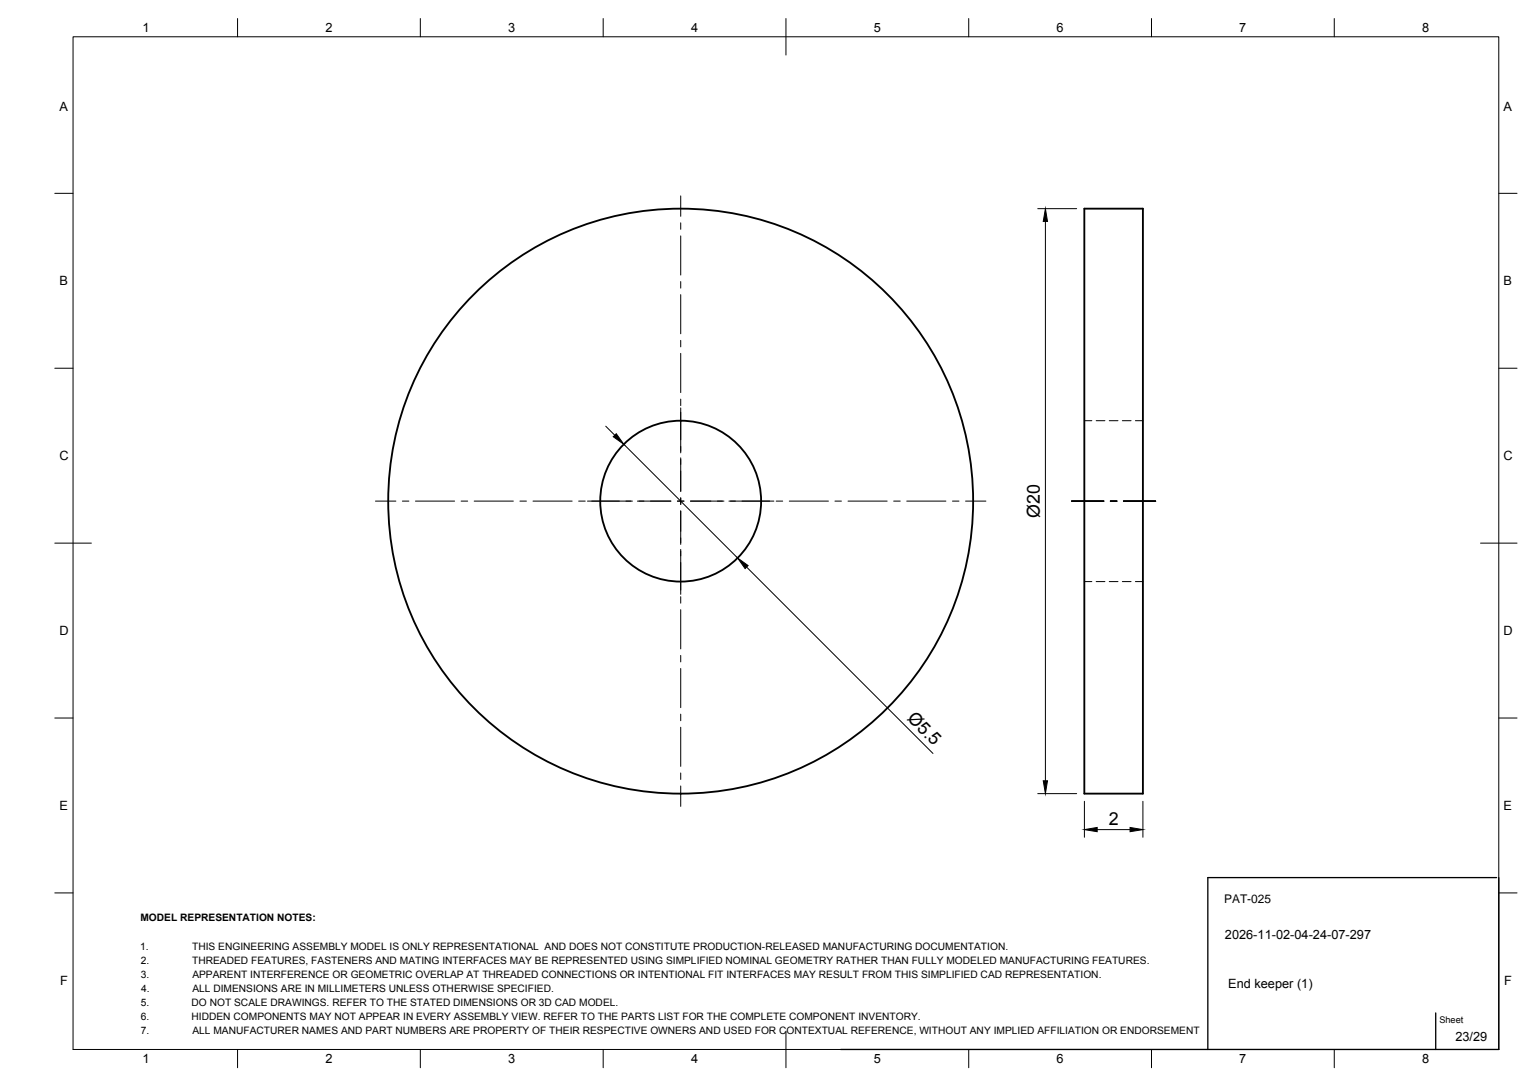
ISO-10303-21;
HEADER;
/* Generated by software containing ST-Developer
 * from STEP Tools, Inc. (www.steptools.com) 
 */

FILE_DESCRIPTION(
/* description */ ('Counter shaft with two pulleys and keyed hub'),
/* implementation_level */ '2;1');

FILE_NAME(
/* name */ 'End keeper (1).step',
/* time_stamp */ '2026-10-27T10:46:10-07:00',
/* author */ (''),
/* organization */ (''),
/* preprocessor_version */ 'ST-DEVELOPER v20.2',
/* originating_system */ 'Autodesk Translation Framework v15.17.0.0',
/* authorisation */ '');

FILE_SCHEMA (('AUTOMOTIVE_DESIGN { 1 0 10303 214 3 1 1 }'));
ENDSEC;

DATA;
#10=MECHANICAL_DESIGN_GEOMETRIC_PRESENTATION_REPRESENTATION('',(#307),#10821);
#256=SHAPE_REPRESENTATION_RELATIONSHIP('SRR','None',#10944,#281);
#281=ADVANCED_BREP_SHAPE_REPRESENTATION('',(#332),#10812);
#307=STYLED_ITEM('',(#11149),#332);
#332=MANIFOLD_SOLID_BREP('Body1',#5591);
#403=FACE_BOUND('',#1109,.T.);
#404=FACE_BOUND('',#1111,.T.);
#523=PLANE('',#6157);
#524=PLANE('',#6158);
#729=FACE_OUTER_BOUND('',#1106,.T.);
#730=FACE_OUTER_BOUND('',#1107,.T.);
#731=FACE_OUTER_BOUND('',#1108,.T.);
#732=FACE_OUTER_BOUND('',#1110,.T.);
#1106=EDGE_LOOP('',(#4207,#4208,#4209,#4210));
#1107=EDGE_LOOP('',(#4211,#4212,#4213,#4214));
#1108=EDGE_LOOP('',(#4215));
#1109=EDGE_LOOP('',(#4216));
#1110=EDGE_LOOP('',(#4217));
#1111=EDGE_LOOP('',(#4218));
#1479=LINE('',#9393,#1868);
#1480=LINE('',#9399,#1869);
#1868=VECTOR('',#7283,0.275);
#1869=VECTOR('',#7290,1.);
#2178=CIRCLE('',#6152,0.275);
#2179=CIRCLE('',#6153,0.275);
#2180=CIRCLE('',#6155,1.);
#2181=CIRCLE('',#6156,1.);
#2583=VERTEX_POINT('',#9390);
#2584=VERTEX_POINT('',#9392);
#2585=VERTEX_POINT('',#9396);
#2586=VERTEX_POINT('',#9398);
#3176=EDGE_CURVE('',#2583,#2583,#2178,.T.);
#3177=EDGE_CURVE('',#2583,#2584,#1479,.T.);
#3178=EDGE_CURVE('',#2584,#2584,#2179,.T.);
#3179=EDGE_CURVE('',#2585,#2585,#2180,.T.);
#3180=EDGE_CURVE('',#2585,#2586,#1480,.T.);
#3181=EDGE_CURVE('',#2586,#2586,#2181,.T.);
#4207=ORIENTED_EDGE('',*,*,#3176,.F.);
#4208=ORIENTED_EDGE('',*,*,#3177,.T.);
#4209=ORIENTED_EDGE('',*,*,#3178,.T.);
#4210=ORIENTED_EDGE('',*,*,#3177,.F.);
#4211=ORIENTED_EDGE('',*,*,#3179,.F.);
#4212=ORIENTED_EDGE('',*,*,#3180,.T.);
#4213=ORIENTED_EDGE('',*,*,#3181,.T.);
#4214=ORIENTED_EDGE('',*,*,#3180,.F.);
#4215=ORIENTED_EDGE('',*,*,#3179,.T.);
#4216=ORIENTED_EDGE('',*,*,#3176,.T.);
#4217=ORIENTED_EDGE('',*,*,#3181,.F.);
#4218=ORIENTED_EDGE('',*,*,#3178,.F.);
#5157=CYLINDRICAL_SURFACE('',#6151,0.275);
#5158=CYLINDRICAL_SURFACE('',#6154,1.);
#5400=ADVANCED_FACE('',(#729),#5157,.F.);
#5401=ADVANCED_FACE('',(#730),#5158,.T.);
#5402=ADVANCED_FACE('',(#731,#403),#523,.T.);
#5403=ADVANCED_FACE('',(#732,#404),#524,.F.);
#5591=CLOSED_SHELL('',(#5400,#5401,#5402,#5403));
#6150=AXIS2_PLACEMENT_3D('',#9388,#7277,#7278);
#6151=AXIS2_PLACEMENT_3D('',#9389,#7279,#7280);
#6152=AXIS2_PLACEMENT_3D('',#9391,#7281,#7282);
#6153=AXIS2_PLACEMENT_3D('',#9394,#7284,#7285);
#6154=AXIS2_PLACEMENT_3D('',#9395,#7286,#7287);
#6155=AXIS2_PLACEMENT_3D('',#9397,#7288,#7289);
#6156=AXIS2_PLACEMENT_3D('',#9400,#7291,#7292);
#6157=AXIS2_PLACEMENT_3D('',#9401,#7293,#7294);
#6158=AXIS2_PLACEMENT_3D('',#9402,#7295,#7296);
#7277=DIRECTION('axis',(0.,0.,1.));
#7278=DIRECTION('refdir',(1.,0.,0.));
#7279=DIRECTION('center_axis',(0.,1.,0.));
#7280=DIRECTION('ref_axis',(1.,0.,0.));
#7281=DIRECTION('center_axis',(0.,-1.,0.));
#7282=DIRECTION('ref_axis',(1.,0.,0.));
#7283=DIRECTION('',(0.,-1.,0.));
#7284=DIRECTION('center_axis',(0.,-1.,0.));
#7285=DIRECTION('ref_axis',(1.,0.,0.));
#7286=DIRECTION('center_axis',(0.,1.,0.));
#7287=DIRECTION('ref_axis',(1.,0.,0.));
#7288=DIRECTION('center_axis',(0.,1.,0.));
#7289=DIRECTION('ref_axis',(1.,0.,0.));
#7290=DIRECTION('',(0.,-1.,0.));
#7291=DIRECTION('center_axis',(0.,1.,0.));
#7292=DIRECTION('ref_axis',(1.,0.,0.));
#7293=DIRECTION('center_axis',(0.,1.,0.));
#7294=DIRECTION('ref_axis',(1.,0.,0.));
#7295=DIRECTION('center_axis',(0.,1.,0.));
#7296=DIRECTION('ref_axis',(1.,0.,0.));
#9388=CARTESIAN_POINT('',(0.,0.,0.));
#9389=CARTESIAN_POINT('Origin',(0.,27.,4.53));
#9390=CARTESIAN_POINT('',(-0.275,27.2,4.53));
#9391=CARTESIAN_POINT('Origin',(0.,27.2,4.53));
#9392=CARTESIAN_POINT('',(-0.275,27.,4.53));
#9393=CARTESIAN_POINT('',(-0.275,27.,4.53));
#9394=CARTESIAN_POINT('Origin',(0.,27.,4.53));
#9395=CARTESIAN_POINT('Origin',(0.,27.,4.53));
#9396=CARTESIAN_POINT('',(-1.,27.2,4.53));
#9397=CARTESIAN_POINT('Origin',(0.,27.2,4.53));
#9398=CARTESIAN_POINT('',(-1.,27.,4.53));
#9399=CARTESIAN_POINT('',(-1.,27.,4.53));
#9400=CARTESIAN_POINT('Origin',(0.,27.,4.53));
#9401=CARTESIAN_POINT('Origin',(0.,27.2,4.53));
#9402=CARTESIAN_POINT('Origin',(0.,27.,4.53));
#10782=UNCERTAINTY_MEASURE_WITH_UNIT(LENGTH_MEASURE(0.001),#10822,
'DISTANCE_ACCURACY_VALUE',
'Maximum model space distance between geometric entities at asserted c
onnectivities');
#10791=UNCERTAINTY_MEASURE_WITH_UNIT(LENGTH_MEASURE(0.001),#10822,
'DISTANCE_ACCURACY_VALUE',
'Maximum model space distance between geometric entities at asserted c
onnectivities');
#10812=(
GEOMETRIC_REPRESENTATION_CONTEXT(3)
GLOBAL_UNCERTAINTY_ASSIGNED_CONTEXT((#10782))
GLOBAL_UNIT_ASSIGNED_CONTEXT((#10822,#10824,#10825))
REPRESENTATION_CONTEXT('','3D')
);
#10821=(
GEOMETRIC_REPRESENTATION_CONTEXT(3)
GLOBAL_UNCERTAINTY_ASSIGNED_CONTEXT((#10791))
GLOBAL_UNIT_ASSIGNED_CONTEXT((#10822,#10824,#10825))
REPRESENTATION_CONTEXT('','3D')
);
#10822=(
LENGTH_UNIT()
NAMED_UNIT(*)
SI_UNIT(.CENTI.,.METRE.)
);
#10824=(
NAMED_UNIT(*)
PLANE_ANGLE_UNIT()
SI_UNIT($,.RADIAN.)
);
#10825=(
NAMED_UNIT(*)
SI_UNIT($,.STERADIAN.)
SOLID_ANGLE_UNIT()
);
#10846=SHAPE_DEFINITION_REPRESENTATION(#10894,#10944);
#10894=PRODUCT_DEFINITION_SHAPE('',$,#10974);
#10944=SHAPE_REPRESENTATION('',(#6150),#10812);
#10953=PRODUCT_DEFINITION_CONTEXT('part definition',#11042,'design');
#10974=PRODUCT_DEFINITION('End keeper (1)','End keeper (1)',#11003,#10953);
#11003=PRODUCT_DEFINITION_FORMATION('',$,#11064);
#11042=APPLICATION_CONTEXT(
'Core Data for Automotive Mechanical Design Process');
#11043=PRODUCT_CONTEXT('part definition',#11042,'mechanical');
#11064=PRODUCT('End keeper (1)','End keeper (1)','End keeper (1)',(#11043));
#11143=COLOUR_RGB('Off White',0.89,0.88,0.83);
#11144=FILL_AREA_STYLE_COLOUR('',#11143);
#11145=FILL_AREA_STYLE('',(#11144));
#11146=SURFACE_STYLE_FILL_AREA(#11145);
#11147=SURFACE_SIDE_STYLE('',(#11146));
#11148=SURFACE_STYLE_USAGE(.BOTH.,#11147);
#11149=PRESENTATION_STYLE_ASSIGNMENT((#11148));
ENDSEC;
END-ISO-10303-21;
